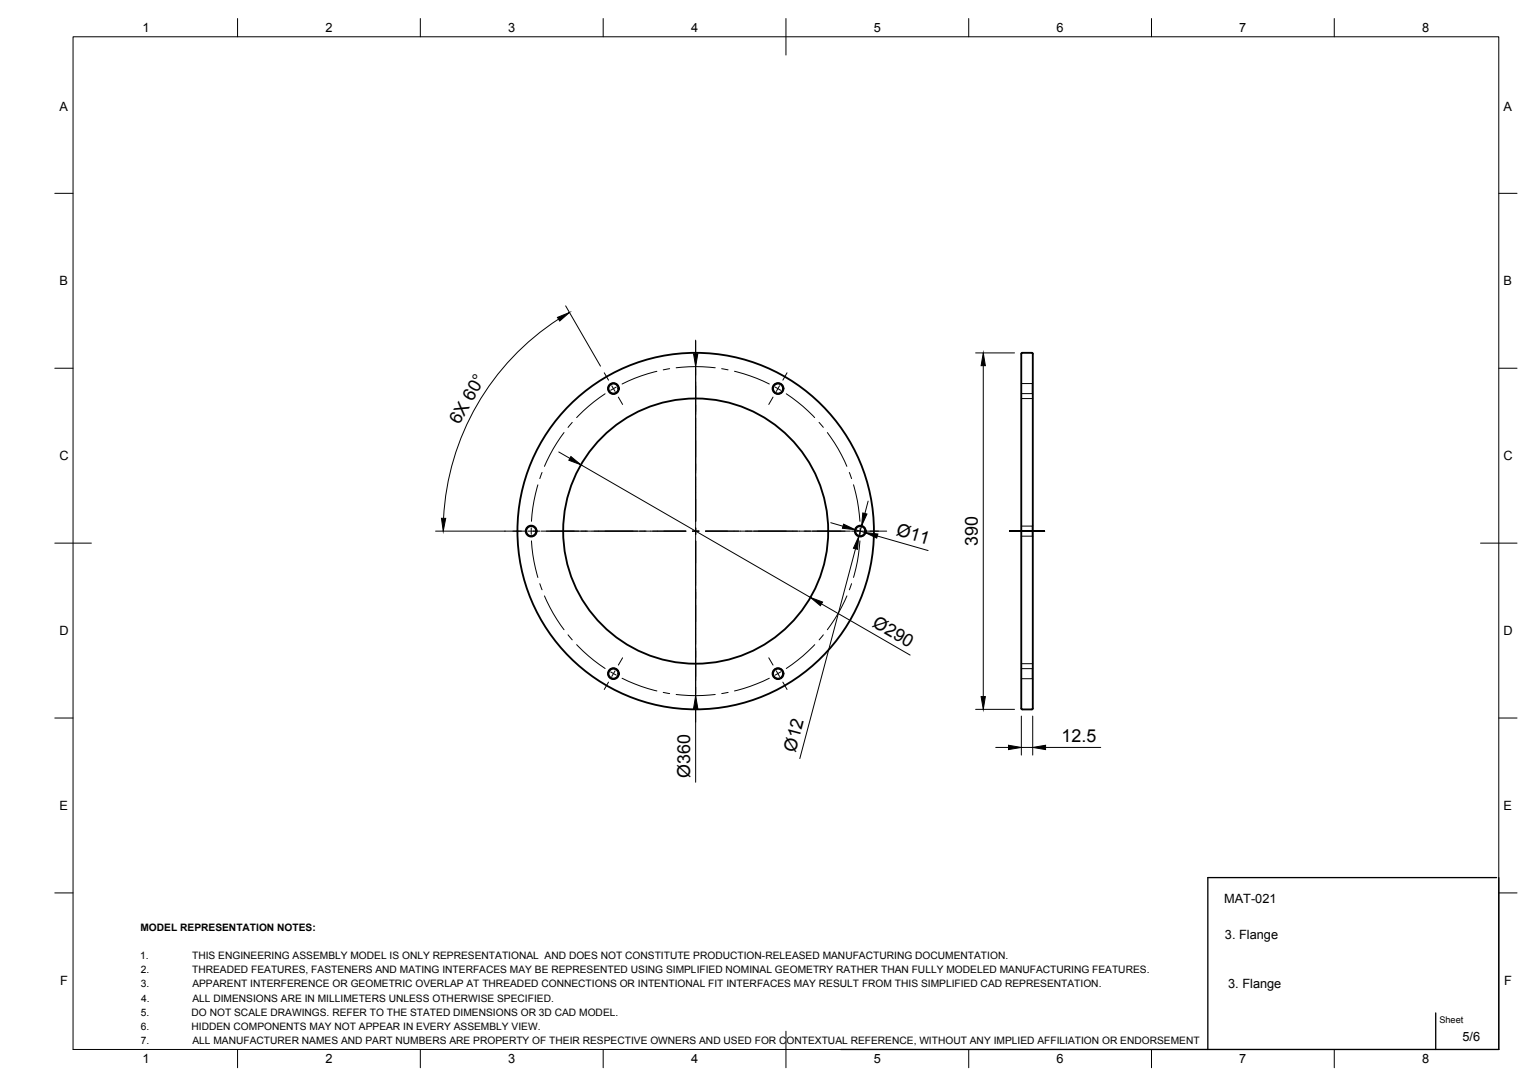
ISO-10303-21;
HEADER;
/* Generated by software containing ST-Developer
 * from STEP Tools, Inc. (www.steptools.com) 
 */

FILE_DESCRIPTION(
/* description */ ('STEP AP214'),
/* implementation_level */ '2;1');

FILE_NAME(
/* name */ '3. Flange.step',
/* time_stamp */ '2026-11-14T06:27:21-08:00',
/* author */ (''),
/* organization */ (''),
/* preprocessor_version */ 'ST-DEVELOPER v20.2',
/* originating_system */ 'Autodesk Translation Framework v15.17.0.0',
/* authorisation */ '');

FILE_SCHEMA (('AUTOMOTIVE_DESIGN { 1 0 10303 214 3 1 1 }'));
ENDSEC;

DATA;
#10=MECHANICAL_DESIGN_GEOMETRIC_PRESENTATION_REPRESENTATION('',(#37),#27541);
#29=SHAPE_REPRESENTATION_RELATIONSHIP('SRR','None',#27563,#33);
#33=ADVANCED_BREP_SHAPE_REPRESENTATION('',(#64),#27539);
#37=STYLED_ITEM('',(#27592),#64);
#64=MANIFOLD_SOLID_BREP('Body1',#11825);
#316=PLANE('',#12664);
#317=PLANE('',#12665);
#583=FACE_BOUND('',#1787,.T.);
#584=FACE_BOUND('',#1788,.T.);
#585=FACE_BOUND('',#1789,.T.);
#586=FACE_BOUND('',#1790,.T.);
#587=FACE_BOUND('',#1791,.T.);
#588=FACE_BOUND('',#1792,.T.);
#589=FACE_BOUND('',#1793,.T.);
#590=FACE_BOUND('',#1795,.T.);
#591=FACE_BOUND('',#1796,.T.);
#592=FACE_BOUND('',#1797,.T.);
#593=FACE_BOUND('',#1798,.T.);
#594=FACE_BOUND('',#1799,.T.);
#595=FACE_BOUND('',#1800,.T.);
#596=FACE_BOUND('',#1801,.T.);
#628=CONICAL_SURFACE('',#12630,6.00000000000001,0.785398163397452);
#629=CONICAL_SURFACE('',#12635,6.00000000000001,0.785398163397452);
#630=CONICAL_SURFACE('',#12640,6.,0.785398163397453);
#631=CONICAL_SURFACE('',#12645,6.00000000000001,0.785398163397452);
#632=CONICAL_SURFACE('',#12650,6.00000000000001,0.785398163397452);
#633=CONICAL_SURFACE('',#12655,6.,0.785398163397453);
#701=TOROIDAL_SURFACE('',#12620,194.,1.);
#702=TOROIDAL_SURFACE('',#12625,194.,1.);
#1048=FACE_OUTER_BOUND('',#1770,.T.);
#1049=FACE_OUTER_BOUND('',#1771,.T.);
#1050=FACE_OUTER_BOUND('',#1772,.T.);
#1051=FACE_OUTER_BOUND('',#1773,.T.);
#1052=FACE_OUTER_BOUND('',#1774,.T.);
#1053=FACE_OUTER_BOUND('',#1775,.T.);
#1054=FACE_OUTER_BOUND('',#1776,.T.);
#1055=FACE_OUTER_BOUND('',#1777,.T.);
#1056=FACE_OUTER_BOUND('',#1778,.T.);
#1057=FACE_OUTER_BOUND('',#1779,.T.);
#1058=FACE_OUTER_BOUND('',#1780,.T.);
#1059=FACE_OUTER_BOUND('',#1781,.T.);
#1060=FACE_OUTER_BOUND('',#1782,.T.);
#1061=FACE_OUTER_BOUND('',#1783,.T.);
#1062=FACE_OUTER_BOUND('',#1784,.T.);
#1063=FACE_OUTER_BOUND('',#1785,.T.);
#1064=FACE_OUTER_BOUND('',#1786,.T.);
#1065=FACE_OUTER_BOUND('',#1794,.T.);
#1770=EDGE_LOOP('',(#9216,#9217,#9218,#9219,#9220));
#1771=EDGE_LOOP('',(#9221,#9222,#9223,#9224,#9225));
#1772=EDGE_LOOP('',(#9226,#9227,#9228,#9229));
#1773=EDGE_LOOP('',(#9230,#9231,#9232,#9233));
#1774=EDGE_LOOP('',(#9234,#9235,#9236,#9237));
#1775=EDGE_LOOP('',(#9238,#9239,#9240,#9241));
#1776=EDGE_LOOP('',(#9242,#9243,#9244,#9245));
#1777=EDGE_LOOP('',(#9246,#9247,#9248,#9249));
#1778=EDGE_LOOP('',(#9250,#9251,#9252,#9253));
#1779=EDGE_LOOP('',(#9254,#9255,#9256,#9257));
#1780=EDGE_LOOP('',(#9258,#9259,#9260,#9261));
#1781=EDGE_LOOP('',(#9262,#9263,#9264,#9265));
#1782=EDGE_LOOP('',(#9266,#9267,#9268,#9269));
#1783=EDGE_LOOP('',(#9270,#9271,#9272,#9273));
#1784=EDGE_LOOP('',(#9274,#9275,#9276,#9277));
#1785=EDGE_LOOP('',(#9278,#9279,#9280,#9281,#9282,#9283));
#1786=EDGE_LOOP('',(#9284));
#1787=EDGE_LOOP('',(#9285));
#1788=EDGE_LOOP('',(#9286));
#1789=EDGE_LOOP('',(#9287));
#1790=EDGE_LOOP('',(#9288));
#1791=EDGE_LOOP('',(#9289));
#1792=EDGE_LOOP('',(#9290));
#1793=EDGE_LOOP('',(#9291));
#1794=EDGE_LOOP('',(#9292));
#1795=EDGE_LOOP('',(#9293));
#1796=EDGE_LOOP('',(#9294));
#1797=EDGE_LOOP('',(#9295));
#1798=EDGE_LOOP('',(#9296));
#1799=EDGE_LOOP('',(#9297));
#1800=EDGE_LOOP('',(#9298));
#1801=EDGE_LOOP('',(#9299));
#2544=CIRCLE('',#12621,194.);
#2545=CIRCLE('',#12622,1.);
#2546=CIRCLE('',#12623,195.);
#2547=CIRCLE('',#12624,195.);
#2548=CIRCLE('',#12626,195.);
#2549=CIRCLE('',#12627,195.);
#2550=CIRCLE('',#12628,1.);
#2551=CIRCLE('',#12629,194.);
#2552=CIRCLE('',#12631,5.50000000000001);
#2553=CIRCLE('',#12632,6.00000000000001);
#2554=CIRCLE('',#12634,5.50000000000001);
#2555=CIRCLE('',#12636,5.50000000000001);
#2556=CIRCLE('',#12637,6.00000000000001);
#2557=CIRCLE('',#12639,5.50000000000001);
#2558=CIRCLE('',#12641,5.5);
#2559=CIRCLE('',#12642,6.);
#2560=CIRCLE('',#12644,5.49999999999999);
#2561=CIRCLE('',#12646,5.50000000000001);
#2562=CIRCLE('',#12647,6.00000000000001);
#2563=CIRCLE('',#12649,5.50000000000001);
#2564=CIRCLE('',#12651,5.50000000000001);
#2565=CIRCLE('',#12652,6.00000000000001);
#2566=CIRCLE('',#12654,5.49999999999998);
#2567=CIRCLE('',#12656,5.5);
#2568=CIRCLE('',#12657,6.);
#2569=CIRCLE('',#12659,5.49999999999999);
#2570=CIRCLE('',#12661,145.);
#2571=CIRCLE('',#12662,145.);
#3120=LINE('',#25791,#4132);
#3121=LINE('',#25796,#4133);
#3122=LINE('',#25801,#4134);
#3123=LINE('',#25806,#4135);
#3124=LINE('',#25811,#4136);
#3125=LINE('',#25816,#4137);
#3126=LINE('',#25821,#4138);
#3127=LINE('',#25826,#4139);
#3128=LINE('',#25831,#4140);
#3129=LINE('',#25836,#4141);
#3130=LINE('',#25841,#4142);
#3131=LINE('',#25846,#4143);
#3132=LINE('',#25851,#4144);
#3133=LINE('',#25854,#4145);
#4132=VECTOR('',#15027,6.00000000000001);
#4133=VECTOR('',#15034,5.50000000000001);
#4134=VECTOR('',#15039,6.00000000000001);
#4135=VECTOR('',#15046,5.50000000000001);
#4136=VECTOR('',#15051,6.);
#4137=VECTOR('',#15058,5.49999999999999);
#4138=VECTOR('',#15063,6.00000000000001);
#4139=VECTOR('',#15070,5.50000000000001);
#4140=VECTOR('',#15075,6.00000000000001);
#4141=VECTOR('',#15082,5.49999999999998);
#4142=VECTOR('',#15087,6.);
#4143=VECTOR('',#15094,5.49999999999999);
#4144=VECTOR('',#15099,145.);
#4145=VECTOR('',#15104,195.);
#5266=VERTEX_POINT('',#25772);
#5267=VERTEX_POINT('',#25774);
#5268=VERTEX_POINT('',#25776);
#5269=VERTEX_POINT('',#25780);
#5270=VERTEX_POINT('',#25781);
#5271=VERTEX_POINT('',#25784);
#5272=VERTEX_POINT('',#25788);
#5273=VERTEX_POINT('',#25790);
#5274=VERTEX_POINT('',#25794);
#5275=VERTEX_POINT('',#25798);
#5276=VERTEX_POINT('',#25800);
#5277=VERTEX_POINT('',#25804);
#5278=VERTEX_POINT('',#25808);
#5279=VERTEX_POINT('',#25810);
#5280=VERTEX_POINT('',#25814);
#5281=VERTEX_POINT('',#25818);
#5282=VERTEX_POINT('',#25820);
#5283=VERTEX_POINT('',#25824);
#5284=VERTEX_POINT('',#25828);
#5285=VERTEX_POINT('',#25830);
#5286=VERTEX_POINT('',#25834);
#5287=VERTEX_POINT('',#25838);
#5288=VERTEX_POINT('',#25840);
#5289=VERTEX_POINT('',#25844);
#5290=VERTEX_POINT('',#25848);
#5291=VERTEX_POINT('',#25850);
#6676=EDGE_CURVE('',#5266,#5266,#2544,.T.);
#6677=EDGE_CURVE('',#5266,#5267,#2545,.T.);
#6678=EDGE_CURVE('',#5268,#5267,#2546,.T.);
#6679=EDGE_CURVE('',#5267,#5268,#2547,.T.);
#6680=EDGE_CURVE('',#5269,#5270,#2548,.T.);
#6681=EDGE_CURVE('',#5270,#5269,#2549,.T.);
#6682=EDGE_CURVE('',#5270,#5271,#2550,.T.);
#6683=EDGE_CURVE('',#5271,#5271,#2551,.T.);
#6684=EDGE_CURVE('',#5272,#5272,#2552,.T.);
#6685=EDGE_CURVE('',#5272,#5273,#3120,.T.);
#6686=EDGE_CURVE('',#5273,#5273,#2553,.T.);
#6687=EDGE_CURVE('',#5274,#5274,#2554,.T.);
#6688=EDGE_CURVE('',#5274,#5272,#3121,.T.);
#6689=EDGE_CURVE('',#5275,#5275,#2555,.T.);
#6690=EDGE_CURVE('',#5275,#5276,#3122,.T.);
#6691=EDGE_CURVE('',#5276,#5276,#2556,.T.);
#6692=EDGE_CURVE('',#5277,#5277,#2557,.T.);
#6693=EDGE_CURVE('',#5277,#5275,#3123,.T.);
#6694=EDGE_CURVE('',#5278,#5278,#2558,.T.);
#6695=EDGE_CURVE('',#5278,#5279,#3124,.T.);
#6696=EDGE_CURVE('',#5279,#5279,#2559,.T.);
#6697=EDGE_CURVE('',#5280,#5280,#2560,.T.);
#6698=EDGE_CURVE('',#5280,#5278,#3125,.T.);
#6699=EDGE_CURVE('',#5281,#5281,#2561,.T.);
#6700=EDGE_CURVE('',#5281,#5282,#3126,.T.);
#6701=EDGE_CURVE('',#5282,#5282,#2562,.T.);
#6702=EDGE_CURVE('',#5283,#5283,#2563,.T.);
#6703=EDGE_CURVE('',#5283,#5281,#3127,.T.);
#6704=EDGE_CURVE('',#5284,#5284,#2564,.T.);
#6705=EDGE_CURVE('',#5284,#5285,#3128,.T.);
#6706=EDGE_CURVE('',#5285,#5285,#2565,.T.);
#6707=EDGE_CURVE('',#5286,#5286,#2566,.T.);
#6708=EDGE_CURVE('',#5286,#5284,#3129,.T.);
#6709=EDGE_CURVE('',#5287,#5287,#2567,.T.);
#6710=EDGE_CURVE('',#5287,#5288,#3130,.T.);
#6711=EDGE_CURVE('',#5288,#5288,#2568,.T.);
#6712=EDGE_CURVE('',#5289,#5289,#2569,.T.);
#6713=EDGE_CURVE('',#5289,#5287,#3131,.T.);
#6714=EDGE_CURVE('',#5290,#5290,#2570,.T.);
#6715=EDGE_CURVE('',#5290,#5291,#3132,.T.);
#6716=EDGE_CURVE('',#5291,#5291,#2571,.T.);
#6717=EDGE_CURVE('',#5269,#5268,#3133,.T.);
#9216=ORIENTED_EDGE('',*,*,#6676,.F.);
#9217=ORIENTED_EDGE('',*,*,#6677,.T.);
#9218=ORIENTED_EDGE('',*,*,#6678,.F.);
#9219=ORIENTED_EDGE('',*,*,#6679,.F.);
#9220=ORIENTED_EDGE('',*,*,#6677,.F.);
#9221=ORIENTED_EDGE('',*,*,#6680,.F.);
#9222=ORIENTED_EDGE('',*,*,#6681,.F.);
#9223=ORIENTED_EDGE('',*,*,#6682,.T.);
#9224=ORIENTED_EDGE('',*,*,#6683,.F.);
#9225=ORIENTED_EDGE('',*,*,#6682,.F.);
#9226=ORIENTED_EDGE('',*,*,#6684,.F.);
#9227=ORIENTED_EDGE('',*,*,#6685,.T.);
#9228=ORIENTED_EDGE('',*,*,#6686,.T.);
#9229=ORIENTED_EDGE('',*,*,#6685,.F.);
#9230=ORIENTED_EDGE('',*,*,#6687,.F.);
#9231=ORIENTED_EDGE('',*,*,#6688,.T.);
#9232=ORIENTED_EDGE('',*,*,#6684,.T.);
#9233=ORIENTED_EDGE('',*,*,#6688,.F.);
#9234=ORIENTED_EDGE('',*,*,#6689,.F.);
#9235=ORIENTED_EDGE('',*,*,#6690,.T.);
#9236=ORIENTED_EDGE('',*,*,#6691,.T.);
#9237=ORIENTED_EDGE('',*,*,#6690,.F.);
#9238=ORIENTED_EDGE('',*,*,#6692,.F.);
#9239=ORIENTED_EDGE('',*,*,#6693,.T.);
#9240=ORIENTED_EDGE('',*,*,#6689,.T.);
#9241=ORIENTED_EDGE('',*,*,#6693,.F.);
#9242=ORIENTED_EDGE('',*,*,#6694,.F.);
#9243=ORIENTED_EDGE('',*,*,#6695,.T.);
#9244=ORIENTED_EDGE('',*,*,#6696,.T.);
#9245=ORIENTED_EDGE('',*,*,#6695,.F.);
#9246=ORIENTED_EDGE('',*,*,#6697,.F.);
#9247=ORIENTED_EDGE('',*,*,#6698,.T.);
#9248=ORIENTED_EDGE('',*,*,#6694,.T.);
#9249=ORIENTED_EDGE('',*,*,#6698,.F.);
#9250=ORIENTED_EDGE('',*,*,#6699,.F.);
#9251=ORIENTED_EDGE('',*,*,#6700,.T.);
#9252=ORIENTED_EDGE('',*,*,#6701,.T.);
#9253=ORIENTED_EDGE('',*,*,#6700,.F.);
#9254=ORIENTED_EDGE('',*,*,#6702,.F.);
#9255=ORIENTED_EDGE('',*,*,#6703,.T.);
#9256=ORIENTED_EDGE('',*,*,#6699,.T.);
#9257=ORIENTED_EDGE('',*,*,#6703,.F.);
#9258=ORIENTED_EDGE('',*,*,#6704,.F.);
#9259=ORIENTED_EDGE('',*,*,#6705,.T.);
#9260=ORIENTED_EDGE('',*,*,#6706,.T.);
#9261=ORIENTED_EDGE('',*,*,#6705,.F.);
#9262=ORIENTED_EDGE('',*,*,#6707,.F.);
#9263=ORIENTED_EDGE('',*,*,#6708,.T.);
#9264=ORIENTED_EDGE('',*,*,#6704,.T.);
#9265=ORIENTED_EDGE('',*,*,#6708,.F.);
#9266=ORIENTED_EDGE('',*,*,#6709,.F.);
#9267=ORIENTED_EDGE('',*,*,#6710,.T.);
#9268=ORIENTED_EDGE('',*,*,#6711,.T.);
#9269=ORIENTED_EDGE('',*,*,#6710,.F.);
#9270=ORIENTED_EDGE('',*,*,#6712,.F.);
#9271=ORIENTED_EDGE('',*,*,#6713,.T.);
#9272=ORIENTED_EDGE('',*,*,#6709,.T.);
#9273=ORIENTED_EDGE('',*,*,#6713,.F.);
#9274=ORIENTED_EDGE('',*,*,#6714,.T.);
#9275=ORIENTED_EDGE('',*,*,#6715,.T.);
#9276=ORIENTED_EDGE('',*,*,#6716,.F.);
#9277=ORIENTED_EDGE('',*,*,#6715,.F.);
#9278=ORIENTED_EDGE('',*,*,#6680,.T.);
#9279=ORIENTED_EDGE('',*,*,#6681,.T.);
#9280=ORIENTED_EDGE('',*,*,#6717,.T.);
#9281=ORIENTED_EDGE('',*,*,#6678,.T.);
#9282=ORIENTED_EDGE('',*,*,#6679,.T.);
#9283=ORIENTED_EDGE('',*,*,#6717,.F.);
#9284=ORIENTED_EDGE('',*,*,#6676,.T.);
#9285=ORIENTED_EDGE('',*,*,#6686,.F.);
#9286=ORIENTED_EDGE('',*,*,#6691,.F.);
#9287=ORIENTED_EDGE('',*,*,#6696,.F.);
#9288=ORIENTED_EDGE('',*,*,#6701,.F.);
#9289=ORIENTED_EDGE('',*,*,#6706,.F.);
#9290=ORIENTED_EDGE('',*,*,#6711,.F.);
#9291=ORIENTED_EDGE('',*,*,#6714,.F.);
#9292=ORIENTED_EDGE('',*,*,#6683,.T.);
#9293=ORIENTED_EDGE('',*,*,#6687,.T.);
#9294=ORIENTED_EDGE('',*,*,#6692,.T.);
#9295=ORIENTED_EDGE('',*,*,#6697,.T.);
#9296=ORIENTED_EDGE('',*,*,#6702,.T.);
#9297=ORIENTED_EDGE('',*,*,#6707,.T.);
#9298=ORIENTED_EDGE('',*,*,#6712,.T.);
#9299=ORIENTED_EDGE('',*,*,#6716,.T.);
#11040=CYLINDRICAL_SURFACE('',#12633,5.50000000000001);
#11041=CYLINDRICAL_SURFACE('',#12638,5.50000000000001);
#11042=CYLINDRICAL_SURFACE('',#12643,5.49999999999999);
#11043=CYLINDRICAL_SURFACE('',#12648,5.50000000000001);
#11044=CYLINDRICAL_SURFACE('',#12653,5.49999999999998);
#11045=CYLINDRICAL_SURFACE('',#12658,5.49999999999999);
#11046=CYLINDRICAL_SURFACE('',#12660,145.);
#11047=CYLINDRICAL_SURFACE('',#12663,195.);
#11487=ADVANCED_FACE('',(#1048),#701,.T.);
#11488=ADVANCED_FACE('',(#1049),#702,.T.);
#11489=ADVANCED_FACE('',(#1050),#628,.F.);
#11490=ADVANCED_FACE('',(#1051),#11040,.F.);
#11491=ADVANCED_FACE('',(#1052),#629,.F.);
#11492=ADVANCED_FACE('',(#1053),#11041,.F.);
#11493=ADVANCED_FACE('',(#1054),#630,.F.);
#11494=ADVANCED_FACE('',(#1055),#11042,.F.);
#11495=ADVANCED_FACE('',(#1056),#631,.F.);
#11496=ADVANCED_FACE('',(#1057),#11043,.F.);
#11497=ADVANCED_FACE('',(#1058),#632,.F.);
#11498=ADVANCED_FACE('',(#1059),#11044,.F.);
#11499=ADVANCED_FACE('',(#1060),#633,.F.);
#11500=ADVANCED_FACE('',(#1061),#11045,.F.);
#11501=ADVANCED_FACE('',(#1062),#11046,.F.);
#11502=ADVANCED_FACE('',(#1063),#11047,.T.);
#11503=ADVANCED_FACE('',(#1064,#583,#584,#585,#586,#587,#588,#589),#316,
 .T.);
#11504=ADVANCED_FACE('',(#1065,#590,#591,#592,#593,#594,#595,#596),#317,
 .F.);
#11825=CLOSED_SHELL('',(#11487,#11488,#11489,#11490,#11491,#11492,#11493,
#11494,#11495,#11496,#11497,#11498,#11499,#11500,#11501,#11502,#11503,#11504));
#12619=AXIS2_PLACEMENT_3D('',#25770,#15001,#15002);
#12620=AXIS2_PLACEMENT_3D('',#25771,#15003,#15004);
#12621=AXIS2_PLACEMENT_3D('',#25773,#15005,#15006);
#12622=AXIS2_PLACEMENT_3D('',#25775,#15007,#15008);
#12623=AXIS2_PLACEMENT_3D('',#25777,#15009,#15010);
#12624=AXIS2_PLACEMENT_3D('',#25778,#15011,#15012);
#12625=AXIS2_PLACEMENT_3D('',#25779,#15013,#15014);
#12626=AXIS2_PLACEMENT_3D('',#25782,#15015,#15016);
#12627=AXIS2_PLACEMENT_3D('',#25783,#15017,#15018);
#12628=AXIS2_PLACEMENT_3D('',#25785,#15019,#15020);
#12629=AXIS2_PLACEMENT_3D('',#25786,#15021,#15022);
#12630=AXIS2_PLACEMENT_3D('',#25787,#15023,#15024);
#12631=AXIS2_PLACEMENT_3D('',#25789,#15025,#15026);
#12632=AXIS2_PLACEMENT_3D('',#25792,#15028,#15029);
#12633=AXIS2_PLACEMENT_3D('',#25793,#15030,#15031);
#12634=AXIS2_PLACEMENT_3D('',#25795,#15032,#15033);
#12635=AXIS2_PLACEMENT_3D('',#25797,#15035,#15036);
#12636=AXIS2_PLACEMENT_3D('',#25799,#15037,#15038);
#12637=AXIS2_PLACEMENT_3D('',#25802,#15040,#15041);
#12638=AXIS2_PLACEMENT_3D('',#25803,#15042,#15043);
#12639=AXIS2_PLACEMENT_3D('',#25805,#15044,#15045);
#12640=AXIS2_PLACEMENT_3D('',#25807,#15047,#15048);
#12641=AXIS2_PLACEMENT_3D('',#25809,#15049,#15050);
#12642=AXIS2_PLACEMENT_3D('',#25812,#15052,#15053);
#12643=AXIS2_PLACEMENT_3D('',#25813,#15054,#15055);
#12644=AXIS2_PLACEMENT_3D('',#25815,#15056,#15057);
#12645=AXIS2_PLACEMENT_3D('',#25817,#15059,#15060);
#12646=AXIS2_PLACEMENT_3D('',#25819,#15061,#15062);
#12647=AXIS2_PLACEMENT_3D('',#25822,#15064,#15065);
#12648=AXIS2_PLACEMENT_3D('',#25823,#15066,#15067);
#12649=AXIS2_PLACEMENT_3D('',#25825,#15068,#15069);
#12650=AXIS2_PLACEMENT_3D('',#25827,#15071,#15072);
#12651=AXIS2_PLACEMENT_3D('',#25829,#15073,#15074);
#12652=AXIS2_PLACEMENT_3D('',#25832,#15076,#15077);
#12653=AXIS2_PLACEMENT_3D('',#25833,#15078,#15079);
#12654=AXIS2_PLACEMENT_3D('',#25835,#15080,#15081);
#12655=AXIS2_PLACEMENT_3D('',#25837,#15083,#15084);
#12656=AXIS2_PLACEMENT_3D('',#25839,#15085,#15086);
#12657=AXIS2_PLACEMENT_3D('',#25842,#15088,#15089);
#12658=AXIS2_PLACEMENT_3D('',#25843,#15090,#15091);
#12659=AXIS2_PLACEMENT_3D('',#25845,#15092,#15093);
#12660=AXIS2_PLACEMENT_3D('',#25847,#15095,#15096);
#12661=AXIS2_PLACEMENT_3D('',#25849,#15097,#15098);
#12662=AXIS2_PLACEMENT_3D('',#25852,#15100,#15101);
#12663=AXIS2_PLACEMENT_3D('',#25853,#15102,#15103);
#12664=AXIS2_PLACEMENT_3D('',#25855,#15105,#15106);
#12665=AXIS2_PLACEMENT_3D('',#25856,#15107,#15108);
#15001=DIRECTION('axis',(0.,0.,1.));
#15002=DIRECTION('refdir',(1.,0.,0.));
#15003=DIRECTION('center_axis',(0.,0.,1.));
#15004=DIRECTION('ref_axis',(1.,0.,0.));
#15005=DIRECTION('center_axis',(0.,0.,1.));
#15006=DIRECTION('ref_axis',(1.,0.,0.));
#15007=DIRECTION('center_axis',(1.22464679914735E-16,-1.,0.));
#15008=DIRECTION('ref_axis',(-1.,-1.22464679914735E-16,0.));
#15009=DIRECTION('center_axis',(0.,0.,-1.));
#15010=DIRECTION('ref_axis',(1.,0.,0.));
#15011=DIRECTION('center_axis',(0.,0.,-1.));
#15012=DIRECTION('ref_axis',(1.,0.,0.));
#15013=DIRECTION('center_axis',(0.,0.,1.));
#15014=DIRECTION('ref_axis',(1.,0.,0.));
#15015=DIRECTION('center_axis',(0.,0.,1.));
#15016=DIRECTION('ref_axis',(1.,0.,0.));
#15017=DIRECTION('center_axis',(0.,0.,1.));
#15018=DIRECTION('ref_axis',(1.,0.,0.));
#15019=DIRECTION('center_axis',(1.22464679914735E-16,-1.,0.));
#15020=DIRECTION('ref_axis',(-1.,-1.22464679914735E-16,0.));
#15021=DIRECTION('center_axis',(0.,0.,-1.));
#15022=DIRECTION('ref_axis',(1.,0.,0.));
#15023=DIRECTION('center_axis',(0.,0.,1.));
#15024=DIRECTION('ref_axis',(1.,0.,0.));
#15025=DIRECTION('center_axis',(0.,0.,1.));
#15026=DIRECTION('ref_axis',(1.,0.,0.));
#15027=DIRECTION('',(-0.70710678118655,-8.65956056235496E-17,0.707106781186545));
#15028=DIRECTION('center_axis',(0.,0.,1.));
#15029=DIRECTION('ref_axis',(1.,0.,0.));
#15030=DIRECTION('center_axis',(0.,0.,1.));
#15031=DIRECTION('ref_axis',(1.,0.,0.));
#15032=DIRECTION('center_axis',(0.,0.,1.));
#15033=DIRECTION('ref_axis',(1.,0.,0.));
#15034=DIRECTION('',(0.,0.,1.));
#15035=DIRECTION('center_axis',(0.,0.,1.));
#15036=DIRECTION('ref_axis',(1.,0.,0.));
#15037=DIRECTION('center_axis',(0.,0.,1.));
#15038=DIRECTION('ref_axis',(1.,0.,0.));
#15039=DIRECTION('',(-0.70710678118655,-8.65956056235496E-17,0.707106781186545));
#15040=DIRECTION('center_axis',(0.,0.,1.));
#15041=DIRECTION('ref_axis',(1.,0.,0.));
#15042=DIRECTION('center_axis',(0.,0.,1.));
#15043=DIRECTION('ref_axis',(1.,0.,0.));
#15044=DIRECTION('center_axis',(0.,0.,1.));
#15045=DIRECTION('ref_axis',(1.,0.,0.));
#15046=DIRECTION('',(0.,0.,1.));
#15047=DIRECTION('center_axis',(0.,0.,1.));
#15048=DIRECTION('ref_axis',(1.,0.,0.));
#15049=DIRECTION('center_axis',(0.,0.,1.));
#15050=DIRECTION('ref_axis',(1.,0.,0.));
#15051=DIRECTION('',(-0.707106781186551,-8.65956056235498E-17,0.707106781186544));
#15052=DIRECTION('center_axis',(0.,0.,1.));
#15053=DIRECTION('ref_axis',(1.,0.,0.));
#15054=DIRECTION('center_axis',(0.,0.,1.));
#15055=DIRECTION('ref_axis',(1.,0.,0.));
#15056=DIRECTION('center_axis',(0.,0.,1.));
#15057=DIRECTION('ref_axis',(1.,0.,0.));
#15058=DIRECTION('',(0.,0.,1.));
#15059=DIRECTION('center_axis',(0.,0.,1.));
#15060=DIRECTION('ref_axis',(1.,0.,0.));
#15061=DIRECTION('center_axis',(0.,0.,1.));
#15062=DIRECTION('ref_axis',(1.,0.,0.));
#15063=DIRECTION('',(-0.70710678118655,-8.65956056235496E-17,0.707106781186545));
#15064=DIRECTION('center_axis',(0.,0.,1.));
#15065=DIRECTION('ref_axis',(1.,0.,0.));
#15066=DIRECTION('center_axis',(0.,0.,1.));
#15067=DIRECTION('ref_axis',(1.,0.,0.));
#15068=DIRECTION('center_axis',(0.,0.,1.));
#15069=DIRECTION('ref_axis',(1.,0.,0.));
#15070=DIRECTION('',(0.,0.,1.));
#15071=DIRECTION('center_axis',(0.,0.,1.));
#15072=DIRECTION('ref_axis',(1.,0.,0.));
#15073=DIRECTION('center_axis',(0.,0.,1.));
#15074=DIRECTION('ref_axis',(1.,0.,0.));
#15075=DIRECTION('',(-0.70710678118655,-8.65956056235496E-17,0.707106781186545));
#15076=DIRECTION('center_axis',(0.,0.,1.));
#15077=DIRECTION('ref_axis',(1.,0.,0.));
#15078=DIRECTION('center_axis',(0.,0.,1.));
#15079=DIRECTION('ref_axis',(1.,0.,0.));
#15080=DIRECTION('center_axis',(0.,0.,1.));
#15081=DIRECTION('ref_axis',(1.,0.,0.));
#15082=DIRECTION('',(0.,0.,1.));
#15083=DIRECTION('center_axis',(0.,0.,1.));
#15084=DIRECTION('ref_axis',(1.,0.,0.));
#15085=DIRECTION('center_axis',(0.,0.,1.));
#15086=DIRECTION('ref_axis',(1.,0.,0.));
#15087=DIRECTION('',(-0.707106781186551,-8.65956056235498E-17,0.707106781186544));
#15088=DIRECTION('center_axis',(0.,0.,1.));
#15089=DIRECTION('ref_axis',(1.,0.,0.));
#15090=DIRECTION('center_axis',(0.,0.,1.));
#15091=DIRECTION('ref_axis',(1.,0.,0.));
#15092=DIRECTION('center_axis',(0.,0.,1.));
#15093=DIRECTION('ref_axis',(1.,0.,0.));
#15094=DIRECTION('',(0.,0.,1.));
#15095=DIRECTION('center_axis',(0.,0.,-1.));
#15096=DIRECTION('ref_axis',(-1.,0.,0.));
#15097=DIRECTION('center_axis',(0.,0.,1.));
#15098=DIRECTION('ref_axis',(1.,0.,0.));
#15099=DIRECTION('',(0.,0.,-1.));
#15100=DIRECTION('center_axis',(0.,0.,1.));
#15101=DIRECTION('ref_axis',(1.,0.,0.));
#15102=DIRECTION('center_axis',(0.,0.,-1.));
#15103=DIRECTION('ref_axis',(-1.,0.,0.));
#15104=DIRECTION('',(0.,0.,1.));
#15105=DIRECTION('center_axis',(0.,0.,1.));
#15106=DIRECTION('ref_axis',(1.,0.,0.));
#15107=DIRECTION('center_axis',(0.,0.,1.));
#15108=DIRECTION('ref_axis',(1.,0.,0.));
#25770=CARTESIAN_POINT('',(0.,0.,0.));
#25771=CARTESIAN_POINT('Origin',(0.,0.,11.5));
#25772=CARTESIAN_POINT('',(-194.,-2.37581479034587E-14,12.5));
#25773=CARTESIAN_POINT('Origin',(0.,0.,12.5));
#25774=CARTESIAN_POINT('',(-195.,-2.38806125833734E-14,11.5));
#25775=CARTESIAN_POINT('Origin',(-194.,-2.37581479034587E-14,11.5));
#25776=CARTESIAN_POINT('',(195.,2.38806125833734E-14,11.5));
#25777=CARTESIAN_POINT('Origin',(0.,0.,11.5));
#25778=CARTESIAN_POINT('Origin',(0.,0.,11.5));
#25779=CARTESIAN_POINT('Origin',(0.,0.,1.));
#25780=CARTESIAN_POINT('',(195.,2.38806125833734E-14,1.));
#25781=CARTESIAN_POINT('',(-195.,-2.38806125833734E-14,1.));
#25782=CARTESIAN_POINT('Origin',(0.,0.,1.));
#25783=CARTESIAN_POINT('Origin',(0.,0.,1.));
#25784=CARTESIAN_POINT('',(-194.,-2.37581479034587E-14,0.));
#25785=CARTESIAN_POINT('Origin',(-194.,-2.37581479034587E-14,1.));
#25786=CARTESIAN_POINT('Origin',(0.,0.,0.));
#25787=CARTESIAN_POINT('Origin',(155.884572681198,90.0000000000018,12.5));
#25788=CARTESIAN_POINT('',(150.384572681198,90.0000000000018,12.));
#25789=CARTESIAN_POINT('Origin',(155.884572681198,90.0000000000018,12.));
#25790=CARTESIAN_POINT('',(149.884572681198,90.0000000000018,12.5));
#25791=CARTESIAN_POINT('',(149.884572681198,90.0000000000018,12.5));
#25792=CARTESIAN_POINT('Origin',(155.884572681198,90.0000000000018,12.5));
#25793=CARTESIAN_POINT('Origin',(155.884572681198,90.0000000000018,12.5));
#25794=CARTESIAN_POINT('',(150.384572681198,90.0000000000018,0.));
#25795=CARTESIAN_POINT('Origin',(155.884572681198,90.0000000000018,0.));
#25796=CARTESIAN_POINT('',(150.384572681198,90.0000000000018,12.5));
#25797=CARTESIAN_POINT('Origin',(155.8845726812,-89.9999999999986,12.5));
#25798=CARTESIAN_POINT('',(150.3845726812,-89.9999999999986,12.));
#25799=CARTESIAN_POINT('Origin',(155.8845726812,-89.9999999999986,12.));
#25800=CARTESIAN_POINT('',(149.8845726812,-89.9999999999986,12.5));
#25801=CARTESIAN_POINT('',(149.8845726812,-89.9999999999986,12.5));
#25802=CARTESIAN_POINT('Origin',(155.8845726812,-89.9999999999986,12.5));
#25803=CARTESIAN_POINT('Origin',(155.8845726812,-89.9999999999986,12.5));
#25804=CARTESIAN_POINT('',(150.3845726812,-89.9999999999986,0.));
#25805=CARTESIAN_POINT('Origin',(155.8845726812,-89.9999999999986,0.));
#25806=CARTESIAN_POINT('',(150.3845726812,-89.9999999999986,12.5));
#25807=CARTESIAN_POINT('Origin',(0.,-180.,12.5));
#25808=CARTESIAN_POINT('',(-5.5,-180.,12.));
#25809=CARTESIAN_POINT('Origin',(0.,-180.,12.));
#25810=CARTESIAN_POINT('',(-6.,-180.,12.5));
#25811=CARTESIAN_POINT('',(-6.,-180.,12.5));
#25812=CARTESIAN_POINT('Origin',(0.,-180.,12.5));
#25813=CARTESIAN_POINT('Origin',(0.,-180.,12.5));
#25814=CARTESIAN_POINT('',(-5.49999999999999,-180.,0.));
#25815=CARTESIAN_POINT('Origin',(0.,-180.,0.));
#25816=CARTESIAN_POINT('',(-5.49999999999999,-180.,12.5));
#25817=CARTESIAN_POINT('Origin',(-155.884572681199,-90.0000000000007,12.5));
#25818=CARTESIAN_POINT('',(-161.384572681199,-90.0000000000007,12.));
#25819=CARTESIAN_POINT('Origin',(-155.884572681199,-90.0000000000007,12.));
#25820=CARTESIAN_POINT('',(-161.884572681199,-90.0000000000007,12.5));
#25821=CARTESIAN_POINT('',(-161.884572681199,-90.0000000000007,12.5));
#25822=CARTESIAN_POINT('Origin',(-155.884572681199,-90.0000000000007,12.5));
#25823=CARTESIAN_POINT('Origin',(-155.884572681199,-90.0000000000007,12.5));
#25824=CARTESIAN_POINT('',(-161.384572681199,-90.0000000000007,0.));
#25825=CARTESIAN_POINT('Origin',(-155.884572681199,-90.0000000000007,0.));
#25826=CARTESIAN_POINT('',(-161.384572681199,-90.0000000000007,12.5));
#25827=CARTESIAN_POINT('Origin',(-155.884572681199,89.9999999999996,12.5));
#25828=CARTESIAN_POINT('',(-161.384572681199,89.9999999999996,12.));
#25829=CARTESIAN_POINT('Origin',(-155.884572681199,89.9999999999996,12.));
#25830=CARTESIAN_POINT('',(-161.884572681199,89.9999999999996,12.5));
#25831=CARTESIAN_POINT('',(-161.884572681199,89.9999999999996,12.5));
#25832=CARTESIAN_POINT('Origin',(-155.884572681199,89.9999999999996,12.5));
#25833=CARTESIAN_POINT('Origin',(-155.884572681199,89.9999999999996,12.5));
#25834=CARTESIAN_POINT('',(-161.384572681199,89.9999999999996,0.));
#25835=CARTESIAN_POINT('Origin',(-155.884572681199,89.9999999999996,0.));
#25836=CARTESIAN_POINT('',(-161.384572681199,89.9999999999996,12.5));
#25837=CARTESIAN_POINT('Origin',(0.,180.,12.5));
#25838=CARTESIAN_POINT('',(-5.5,180.,12.));
#25839=CARTESIAN_POINT('Origin',(0.,180.,12.));
#25840=CARTESIAN_POINT('',(-6.,180.,12.5));
#25841=CARTESIAN_POINT('',(-6.,180.,12.5));
#25842=CARTESIAN_POINT('Origin',(0.,180.,12.5));
#25843=CARTESIAN_POINT('Origin',(0.,180.,12.5));
#25844=CARTESIAN_POINT('',(-5.49999999999999,180.,0.));
#25845=CARTESIAN_POINT('Origin',(0.,180.,0.));
#25846=CARTESIAN_POINT('',(-5.49999999999999,180.,12.5));
#25847=CARTESIAN_POINT('Origin',(0.,0.,12.5));
#25848=CARTESIAN_POINT('',(145.,-1.77573785876366E-14,12.5));
#25849=CARTESIAN_POINT('Origin',(0.,0.,12.5));
#25850=CARTESIAN_POINT('',(145.,-1.77573785876366E-14,0.));
#25851=CARTESIAN_POINT('',(145.,-1.77573785876366E-14,12.5));
#25852=CARTESIAN_POINT('Origin',(0.,0.,0.));
#25853=CARTESIAN_POINT('Origin',(0.,0.,12.5));
#25854=CARTESIAN_POINT('',(195.,-2.38806125833734E-14,12.5));
#25855=CARTESIAN_POINT('Origin',(0.,0.,12.5));
#25856=CARTESIAN_POINT('Origin',(0.,0.,0.));
#27533=UNCERTAINTY_MEASURE_WITH_UNIT(LENGTH_MEASURE(0.01),#27542,
'DISTANCE_ACCURACY_VALUE',
'Maximum model space distance between geometric entities at asserted c
onnectivities');
#27535=UNCERTAINTY_MEASURE_WITH_UNIT(LENGTH_MEASURE(0.01),#27542,
'DISTANCE_ACCURACY_VALUE',
'Maximum model space distance between geometric entities at asserted c
onnectivities');
#27539=(
GEOMETRIC_REPRESENTATION_CONTEXT(3)
GLOBAL_UNCERTAINTY_ASSIGNED_CONTEXT((#27533))
GLOBAL_UNIT_ASSIGNED_CONTEXT((#27542,#27544,#27545))
REPRESENTATION_CONTEXT('','3D')
);
#27541=(
GEOMETRIC_REPRESENTATION_CONTEXT(3)
GLOBAL_UNCERTAINTY_ASSIGNED_CONTEXT((#27535))
GLOBAL_UNIT_ASSIGNED_CONTEXT((#27542,#27544,#27545))
REPRESENTATION_CONTEXT('','3D')
);
#27542=(
LENGTH_UNIT()
NAMED_UNIT(*)
SI_UNIT(.MILLI.,.METRE.)
);
#27544=(
NAMED_UNIT(*)
PLANE_ANGLE_UNIT()
SI_UNIT($,.RADIAN.)
);
#27545=(
NAMED_UNIT(*)
SI_UNIT($,.STERADIAN.)
SOLID_ANGLE_UNIT()
);
#27549=SHAPE_DEFINITION_REPRESENTATION(#27554,#27563);
#27554=PRODUCT_DEFINITION_SHAPE('',$,#27569);
#27563=SHAPE_REPRESENTATION('',(#12619),#27539);
#27565=PRODUCT_DEFINITION_CONTEXT('part definition',#27582,'design');
#27569=PRODUCT_DEFINITION('3. Flange','3. Flange',#27574,#27565);
#27574=PRODUCT_DEFINITION_FORMATION('',$,#27587);
#27582=APPLICATION_CONTEXT(
'Core Data for Automotive Mechanical Design Process');
#27583=PRODUCT_CONTEXT('part definition',#27582,'mechanical');
#27587=PRODUCT('3. Flange','3. Flange',$,(#27583));
#27592=PRESENTATION_STYLE_ASSIGNMENT((#27596));
#27596=SURFACE_STYLE_USAGE(.BOTH.,#27600);
#27600=SURFACE_SIDE_STYLE('',(#27604));
#27604=SURFACE_STYLE_FILL_AREA(#27608);
#27608=FILL_AREA_STYLE('Opaque(97,158,199)',(#27612));
#27612=FILL_AREA_STYLE_COLOUR('Opaque(97,158,199)',#27616);
#27616=COLOUR_RGB('Opaque(97,158,199)',0.380392156862745,0.619607843137255,
0.780392156862745);
ENDSEC;
END-ISO-10303-21;
